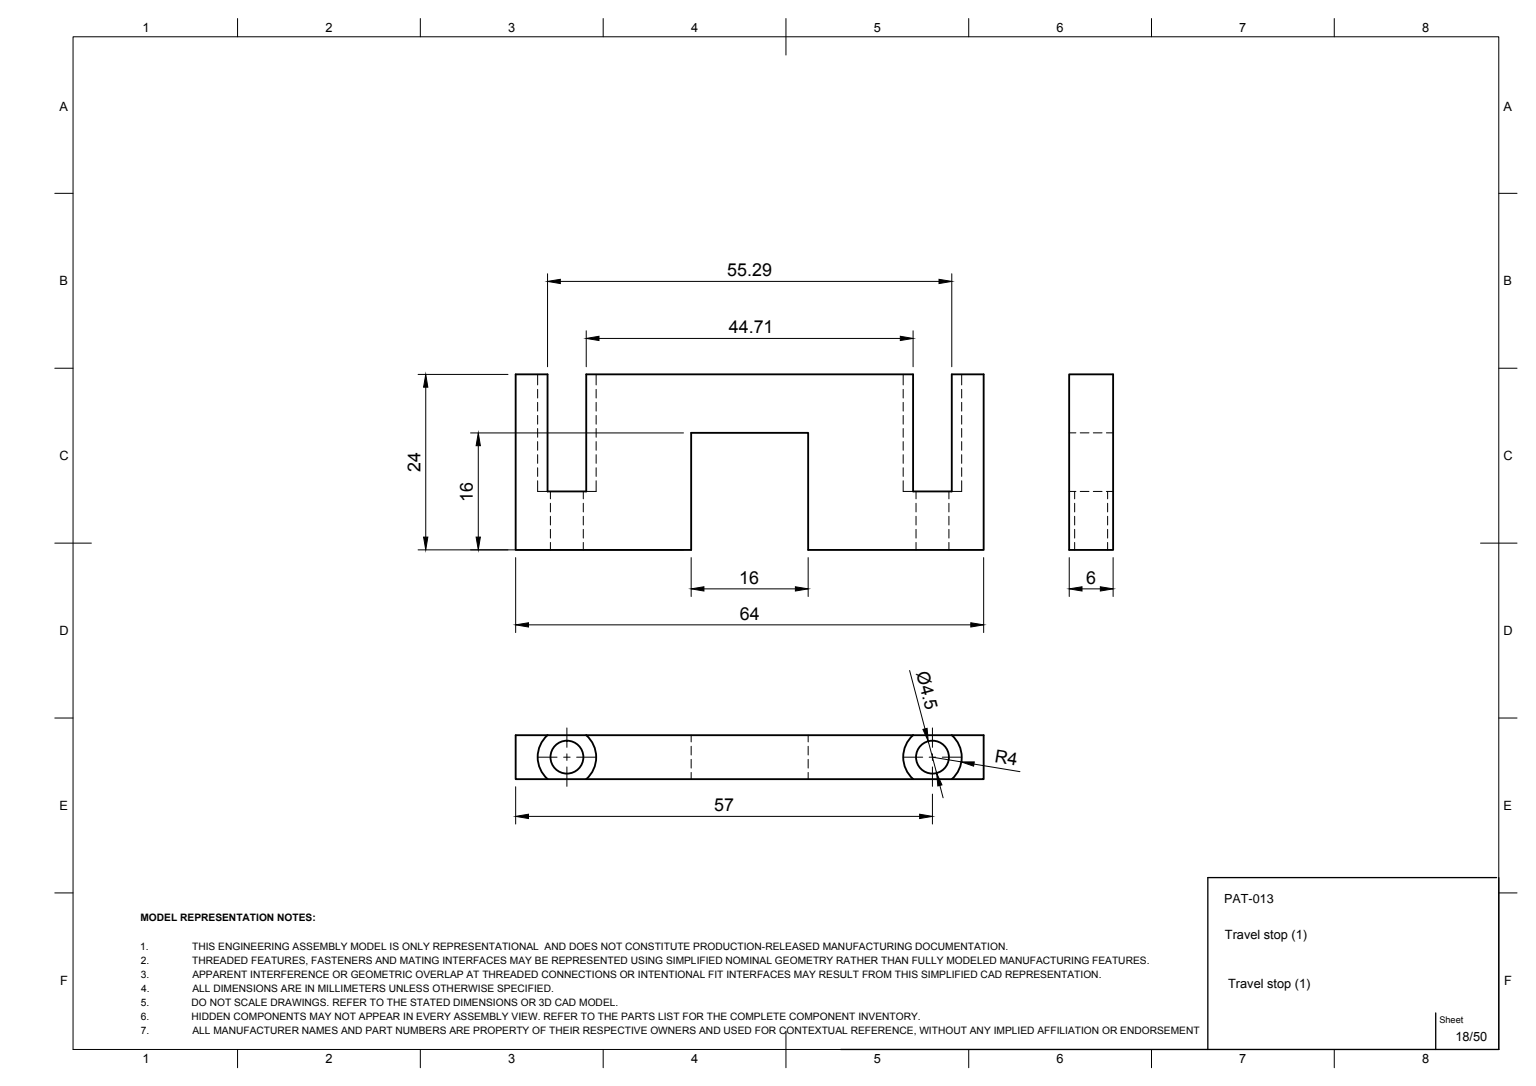
ISO-10303-21;
HEADER;
/* Generated by software containing ST-Developer
 * from STEP Tools, Inc. (www.steptools.com) 
 */

FILE_DESCRIPTION(
/* description */ ('Belt-driven linear axis on 2020 extrusion'),
/* implementation_level */ '2;1');

FILE_NAME(
/* name */ 'Travel stop (1).step',
/* time_stamp */ '2026-10-28T03:26:09-07:00',
/* author */ (''),
/* organization */ (''),
/* preprocessor_version */ 'ST-DEVELOPER v20.2',
/* originating_system */ 'Autodesk Translation Framework v15.17.0.0',
/* authorisation */ '');

FILE_SCHEMA (('AUTOMOTIVE_DESIGN { 1 0 10303 214 3 1 1 }'));
ENDSEC;

DATA;
#10=MECHANICAL_DESIGN_GEOMETRIC_PRESENTATION_REPRESENTATION('',(#625),#20096);
#531=SHAPE_REPRESENTATION_RELATIONSHIP('SRR','None',#20327,#577);
#577=ADVANCED_BREP_SHAPE_REPRESENTATION('',(#681),#20058);
#625=STYLED_ITEM('',(#20636),#681);
#681=MANIFOLD_SOLID_BREP('Body1',#10938);
#800=FACE_BOUND('',#2151,.T.);
#801=FACE_BOUND('',#2155,.T.);
#802=FACE_BOUND('',#2167,.T.);
#803=FACE_BOUND('',#2169,.T.);
#991=PLANE('',#11890);
#992=PLANE('',#11898);
#993=PLANE('',#11900);
#994=PLANE('',#11901);
#995=PLANE('',#11902);
#996=PLANE('',#11903);
#997=PLANE('',#11908);
#998=PLANE('',#11909);
#999=PLANE('',#11910);
#1000=PLANE('',#11911);
#1001=PLANE('',#11912);
#1002=PLANE('',#11913);
#1003=PLANE('',#11914);
#1004=PLANE('',#11915);
#1444=FACE_OUTER_BOUND('',#2148,.T.);
#1445=FACE_OUTER_BOUND('',#2149,.T.);
#1446=FACE_OUTER_BOUND('',#2150,.T.);
#1447=FACE_OUTER_BOUND('',#2152,.T.);
#1448=FACE_OUTER_BOUND('',#2153,.T.);
#1449=FACE_OUTER_BOUND('',#2154,.T.);
#1450=FACE_OUTER_BOUND('',#2156,.T.);
#1451=FACE_OUTER_BOUND('',#2157,.T.);
#1452=FACE_OUTER_BOUND('',#2158,.T.);
#1453=FACE_OUTER_BOUND('',#2159,.T.);
#1454=FACE_OUTER_BOUND('',#2160,.T.);
#1455=FACE_OUTER_BOUND('',#2161,.T.);
#1456=FACE_OUTER_BOUND('',#2162,.T.);
#1457=FACE_OUTER_BOUND('',#2163,.T.);
#1458=FACE_OUTER_BOUND('',#2164,.T.);
#1459=FACE_OUTER_BOUND('',#2165,.T.);
#1460=FACE_OUTER_BOUND('',#2166,.T.);
#1461=FACE_OUTER_BOUND('',#2168,.T.);
#1462=FACE_OUTER_BOUND('',#2170,.T.);
#1463=FACE_OUTER_BOUND('',#2171,.T.);
#2148=EDGE_LOOP('',(#8117,#8118,#8119,#8120));
#2149=EDGE_LOOP('',(#8121,#8122,#8123,#8124));
#2150=EDGE_LOOP('',(#8125,#8126,#8127,#8128));
#2151=EDGE_LOOP('',(#8129));
#2152=EDGE_LOOP('',(#8130,#8131,#8132,#8133));
#2153=EDGE_LOOP('',(#8134,#8135,#8136,#8137));
#2154=EDGE_LOOP('',(#8138,#8139,#8140,#8141));
#2155=EDGE_LOOP('',(#8142));
#2156=EDGE_LOOP('',(#8143,#8144,#8145,#8146,#8147,#8148,#8149,#8150,#8151,
#8152,#8153,#8154,#8155,#8156,#8157,#8158));
#2157=EDGE_LOOP('',(#8159,#8160,#8161,#8162));
#2158=EDGE_LOOP('',(#8163,#8164,#8165,#8166));
#2159=EDGE_LOOP('',(#8167,#8168,#8169,#8170));
#2160=EDGE_LOOP('',(#8171,#8172,#8173,#8174));
#2161=EDGE_LOOP('',(#8175,#8176,#8177,#8178));
#2162=EDGE_LOOP('',(#8179,#8180,#8181,#8182));
#2163=EDGE_LOOP('',(#8183,#8184,#8185,#8186));
#2164=EDGE_LOOP('',(#8187,#8188,#8189,#8190));
#2165=EDGE_LOOP('',(#8191,#8192,#8193,#8194,#8195,#8196,#8197,#8198,#8199,
#8200,#8201,#8202,#8203,#8204,#8205,#8206));
#2166=EDGE_LOOP('',(#8207,#8208,#8209,#8210));
#2167=EDGE_LOOP('',(#8211));
#2168=EDGE_LOOP('',(#8212,#8213,#8214,#8215));
#2169=EDGE_LOOP('',(#8216));
#2170=EDGE_LOOP('',(#8217,#8218,#8219,#8220));
#2171=EDGE_LOOP('',(#8221,#8222,#8223,#8224));
#2913=LINE('',#17165,#3770);
#2914=LINE('',#17169,#3771);
#2915=LINE('',#17174,#3772);
#2916=LINE('',#17178,#3773);
#2917=LINE('',#17181,#3774);
#2918=LINE('',#17182,#3775);
#2919=LINE('',#17188,#3776);
#2920=LINE('',#17192,#3777);
#2921=LINE('',#17197,#3778);
#2922=LINE('',#17201,#3779);
#2923=LINE('',#17204,#3780);
#2924=LINE('',#17205,#3781);
#2925=LINE('',#17210,#3782);
#2926=LINE('',#17212,#3783);
#2927=LINE('',#17214,#3784);
#2928=LINE('',#17216,#3785);
#2929=LINE('',#17218,#3786);
#2930=LINE('',#17220,#3787);
#2931=LINE('',#17222,#3788);
#2932=LINE('',#17224,#3789);
#2933=LINE('',#17225,#3790);
#2934=LINE('',#17226,#3791);
#2935=LINE('',#17229,#3792);
#2936=LINE('',#17230,#3793);
#2937=LINE('',#17233,#3794);
#2938=LINE('',#17234,#3795);
#2939=LINE('',#17236,#3796);
#2940=LINE('',#17240,#3797);
#2941=LINE('',#17244,#3798);
#2942=LINE('',#17247,#3799);
#2943=LINE('',#17249,#3800);
#2944=LINE('',#17250,#3801);
#2945=LINE('',#17253,#3802);
#2946=LINE('',#17255,#3803);
#2947=LINE('',#17256,#3804);
#2948=LINE('',#17258,#3805);
#2949=LINE('',#17261,#3806);
#2950=LINE('',#17262,#3807);
#2951=LINE('',#17264,#3808);
#2952=LINE('',#17265,#3809);
#2953=LINE('',#17267,#3810);
#2954=LINE('',#17269,#3811);
#3770=VECTOR('',#13823,1.);
#3771=VECTOR('',#13826,1.);
#3772=VECTOR('',#13831,1.);
#3773=VECTOR('',#13834,1.);
#3774=VECTOR('',#13839,1.);
#3775=VECTOR('',#13840,1.);
#3776=VECTOR('',#13845,1.);
#3777=VECTOR('',#13848,1.);
#3778=VECTOR('',#13853,1.);
#3779=VECTOR('',#13856,1.);
#3780=VECTOR('',#13861,1.);
#3781=VECTOR('',#13862,1.);
#3782=VECTOR('',#13867,1.);
#3783=VECTOR('',#13868,1.);
#3784=VECTOR('',#13869,1.);
#3785=VECTOR('',#13870,1.);
#3786=VECTOR('',#13871,1.);
#3787=VECTOR('',#13872,1.);
#3788=VECTOR('',#13873,1.);
#3789=VECTOR('',#13874,1.);
#3790=VECTOR('',#13875,1.);
#3791=VECTOR('',#13876,1.);
#3792=VECTOR('',#13879,1.);
#3793=VECTOR('',#13880,1.);
#3794=VECTOR('',#13883,1.);
#3795=VECTOR('',#13884,1.);
#3796=VECTOR('',#13887,1.);
#3797=VECTOR('',#13892,0.225000000000001);
#3798=VECTOR('',#13897,0.225000000000001);
#3799=VECTOR('',#13900,1.);
#3800=VECTOR('',#13901,1.);
#3801=VECTOR('',#13902,1.);
#3802=VECTOR('',#13905,1.);
#3803=VECTOR('',#13906,1.);
#3804=VECTOR('',#13907,1.);
#3805=VECTOR('',#13910,1.);
#3806=VECTOR('',#13913,1.);
#3807=VECTOR('',#13914,1.);
#3808=VECTOR('',#13915,1.);
#3809=VECTOR('',#13916,1.);
#3810=VECTOR('',#13919,1.);
#3811=VECTOR('',#13922,1.);
#4563=CIRCLE('',#11885,0.399999999999999);
#4564=CIRCLE('',#11886,0.399999999999999);
#4565=CIRCLE('',#11888,0.399999999999999);
#4566=CIRCLE('',#11889,0.399999999999999);
#4567=CIRCLE('',#11891,0.225000000000001);
#4568=CIRCLE('',#11893,0.399999999999999);
#4569=CIRCLE('',#11894,0.399999999999999);
#4570=CIRCLE('',#11896,0.399999999999999);
#4571=CIRCLE('',#11897,0.399999999999999);
#4572=CIRCLE('',#11899,0.225000000000001);
#4573=CIRCLE('',#11905,0.225000000000001);
#4574=CIRCLE('',#11907,0.225000000000001);
#5180=VERTEX_POINT('',#17163);
#5181=VERTEX_POINT('',#17164);
#5182=VERTEX_POINT('',#17166);
#5183=VERTEX_POINT('',#17168);
#5184=VERTEX_POINT('',#17172);
#5185=VERTEX_POINT('',#17173);
#5186=VERTEX_POINT('',#17175);
#5187=VERTEX_POINT('',#17177);
#5188=VERTEX_POINT('',#17183);
#5189=VERTEX_POINT('',#17186);
#5190=VERTEX_POINT('',#17187);
#5191=VERTEX_POINT('',#17189);
#5192=VERTEX_POINT('',#17191);
#5193=VERTEX_POINT('',#17195);
#5194=VERTEX_POINT('',#17196);
#5195=VERTEX_POINT('',#17198);
#5196=VERTEX_POINT('',#17200);
#5197=VERTEX_POINT('',#17206);
#5198=VERTEX_POINT('',#17209);
#5199=VERTEX_POINT('',#17211);
#5200=VERTEX_POINT('',#17213);
#5201=VERTEX_POINT('',#17215);
#5202=VERTEX_POINT('',#17217);
#5203=VERTEX_POINT('',#17219);
#5204=VERTEX_POINT('',#17221);
#5205=VERTEX_POINT('',#17223);
#5206=VERTEX_POINT('',#17228);
#5207=VERTEX_POINT('',#17232);
#5208=VERTEX_POINT('',#17238);
#5209=VERTEX_POINT('',#17242);
#5210=VERTEX_POINT('',#17246);
#5211=VERTEX_POINT('',#17248);
#5212=VERTEX_POINT('',#17252);
#5213=VERTEX_POINT('',#17254);
#5214=VERTEX_POINT('',#17260);
#5215=VERTEX_POINT('',#17263);
#6273=EDGE_CURVE('',#5180,#5181,#2913,.T.);
#6274=EDGE_CURVE('',#5182,#5180,#4563,.T.);
#6275=EDGE_CURVE('',#5183,#5182,#2914,.T.);
#6276=EDGE_CURVE('',#5181,#5183,#4564,.T.);
#6277=EDGE_CURVE('',#5184,#5185,#2915,.T.);
#6278=EDGE_CURVE('',#5186,#5184,#4565,.T.);
#6279=EDGE_CURVE('',#5187,#5186,#2916,.T.);
#6280=EDGE_CURVE('',#5185,#5187,#4566,.T.);
#6281=EDGE_CURVE('',#5181,#5184,#2917,.T.);
#6282=EDGE_CURVE('',#5186,#5183,#2918,.T.);
#6283=EDGE_CURVE('',#5188,#5188,#4567,.T.);
#6284=EDGE_CURVE('',#5189,#5190,#2919,.T.);
#6285=EDGE_CURVE('',#5191,#5189,#4568,.T.);
#6286=EDGE_CURVE('',#5192,#5191,#2920,.T.);
#6287=EDGE_CURVE('',#5190,#5192,#4569,.T.);
#6288=EDGE_CURVE('',#5193,#5194,#2921,.T.);
#6289=EDGE_CURVE('',#5195,#5193,#4570,.T.);
#6290=EDGE_CURVE('',#5196,#5195,#2922,.T.);
#6291=EDGE_CURVE('',#5194,#5196,#4571,.T.);
#6292=EDGE_CURVE('',#5190,#5193,#2923,.T.);
#6293=EDGE_CURVE('',#5195,#5192,#2924,.T.);
#6294=EDGE_CURVE('',#5197,#5197,#4572,.T.);
#6295=EDGE_CURVE('',#5198,#5182,#2925,.T.);
#6296=EDGE_CURVE('',#5199,#5198,#2926,.T.);
#6297=EDGE_CURVE('',#5199,#5200,#2927,.T.);
#6298=EDGE_CURVE('',#5200,#5201,#2928,.T.);
#6299=EDGE_CURVE('',#5201,#5202,#2929,.T.);
#6300=EDGE_CURVE('',#5202,#5203,#2930,.T.);
#6301=EDGE_CURVE('',#5203,#5204,#2931,.T.);
#6302=EDGE_CURVE('',#5204,#5205,#2932,.T.);
#6303=EDGE_CURVE('',#5196,#5205,#2933,.T.);
#6304=EDGE_CURVE('',#5187,#5191,#2934,.T.);
#6305=EDGE_CURVE('',#5205,#5206,#2935,.T.);
#6306=EDGE_CURVE('',#5206,#5194,#2936,.T.);
#6307=EDGE_CURVE('',#5180,#5207,#2937,.T.);
#6308=EDGE_CURVE('',#5207,#5198,#2938,.T.);
#6309=EDGE_CURVE('',#5189,#5185,#2939,.T.);
#6310=EDGE_CURVE('',#5208,#5208,#4573,.T.);
#6311=EDGE_CURVE('',#5208,#5188,#2940,.T.);
#6312=EDGE_CURVE('',#5209,#5209,#4574,.T.);
#6313=EDGE_CURVE('',#5209,#5197,#2941,.T.);
#6314=EDGE_CURVE('',#5202,#5210,#2942,.T.);
#6315=EDGE_CURVE('',#5211,#5210,#2943,.T.);
#6316=EDGE_CURVE('',#5203,#5211,#2944,.T.);
#6317=EDGE_CURVE('',#5212,#5200,#2945,.T.);
#6318=EDGE_CURVE('',#5213,#5212,#2946,.T.);
#6319=EDGE_CURVE('',#5213,#5201,#2947,.T.);
#6320=EDGE_CURVE('',#5210,#5213,#2948,.T.);
#6321=EDGE_CURVE('',#5214,#5206,#2949,.T.);
#6322=EDGE_CURVE('',#5214,#5211,#2950,.T.);
#6323=EDGE_CURVE('',#5212,#5215,#2951,.T.);
#6324=EDGE_CURVE('',#5215,#5207,#2952,.T.);
#6325=EDGE_CURVE('',#5215,#5199,#2953,.T.);
#6326=EDGE_CURVE('',#5204,#5214,#2954,.T.);
#8117=ORIENTED_EDGE('',*,*,#6273,.F.);
#8118=ORIENTED_EDGE('',*,*,#6274,.F.);
#8119=ORIENTED_EDGE('',*,*,#6275,.F.);
#8120=ORIENTED_EDGE('',*,*,#6276,.F.);
#8121=ORIENTED_EDGE('',*,*,#6277,.F.);
#8122=ORIENTED_EDGE('',*,*,#6278,.F.);
#8123=ORIENTED_EDGE('',*,*,#6279,.F.);
#8124=ORIENTED_EDGE('',*,*,#6280,.F.);
#8125=ORIENTED_EDGE('',*,*,#6281,.F.);
#8126=ORIENTED_EDGE('',*,*,#6276,.T.);
#8127=ORIENTED_EDGE('',*,*,#6282,.F.);
#8128=ORIENTED_EDGE('',*,*,#6278,.T.);
#8129=ORIENTED_EDGE('',*,*,#6283,.F.);
#8130=ORIENTED_EDGE('',*,*,#6284,.F.);
#8131=ORIENTED_EDGE('',*,*,#6285,.F.);
#8132=ORIENTED_EDGE('',*,*,#6286,.F.);
#8133=ORIENTED_EDGE('',*,*,#6287,.F.);
#8134=ORIENTED_EDGE('',*,*,#6288,.F.);
#8135=ORIENTED_EDGE('',*,*,#6289,.F.);
#8136=ORIENTED_EDGE('',*,*,#6290,.F.);
#8137=ORIENTED_EDGE('',*,*,#6291,.F.);
#8138=ORIENTED_EDGE('',*,*,#6292,.F.);
#8139=ORIENTED_EDGE('',*,*,#6287,.T.);
#8140=ORIENTED_EDGE('',*,*,#6293,.F.);
#8141=ORIENTED_EDGE('',*,*,#6289,.T.);
#8142=ORIENTED_EDGE('',*,*,#6294,.F.);
#8143=ORIENTED_EDGE('',*,*,#6279,.T.);
#8144=ORIENTED_EDGE('',*,*,#6282,.T.);
#8145=ORIENTED_EDGE('',*,*,#6275,.T.);
#8146=ORIENTED_EDGE('',*,*,#6295,.F.);
#8147=ORIENTED_EDGE('',*,*,#6296,.F.);
#8148=ORIENTED_EDGE('',*,*,#6297,.T.);
#8149=ORIENTED_EDGE('',*,*,#6298,.T.);
#8150=ORIENTED_EDGE('',*,*,#6299,.T.);
#8151=ORIENTED_EDGE('',*,*,#6300,.T.);
#8152=ORIENTED_EDGE('',*,*,#6301,.T.);
#8153=ORIENTED_EDGE('',*,*,#6302,.T.);
#8154=ORIENTED_EDGE('',*,*,#6303,.F.);
#8155=ORIENTED_EDGE('',*,*,#6290,.T.);
#8156=ORIENTED_EDGE('',*,*,#6293,.T.);
#8157=ORIENTED_EDGE('',*,*,#6286,.T.);
#8158=ORIENTED_EDGE('',*,*,#6304,.F.);
#8159=ORIENTED_EDGE('',*,*,#6291,.T.);
#8160=ORIENTED_EDGE('',*,*,#6303,.T.);
#8161=ORIENTED_EDGE('',*,*,#6305,.T.);
#8162=ORIENTED_EDGE('',*,*,#6306,.T.);
#8163=ORIENTED_EDGE('',*,*,#6274,.T.);
#8164=ORIENTED_EDGE('',*,*,#6307,.T.);
#8165=ORIENTED_EDGE('',*,*,#6308,.T.);
#8166=ORIENTED_EDGE('',*,*,#6295,.T.);
#8167=ORIENTED_EDGE('',*,*,#6280,.T.);
#8168=ORIENTED_EDGE('',*,*,#6304,.T.);
#8169=ORIENTED_EDGE('',*,*,#6285,.T.);
#8170=ORIENTED_EDGE('',*,*,#6309,.T.);
#8171=ORIENTED_EDGE('',*,*,#6310,.F.);
#8172=ORIENTED_EDGE('',*,*,#6311,.T.);
#8173=ORIENTED_EDGE('',*,*,#6283,.T.);
#8174=ORIENTED_EDGE('',*,*,#6311,.F.);
#8175=ORIENTED_EDGE('',*,*,#6312,.F.);
#8176=ORIENTED_EDGE('',*,*,#6313,.T.);
#8177=ORIENTED_EDGE('',*,*,#6294,.T.);
#8178=ORIENTED_EDGE('',*,*,#6313,.F.);
#8179=ORIENTED_EDGE('',*,*,#6300,.F.);
#8180=ORIENTED_EDGE('',*,*,#6314,.T.);
#8181=ORIENTED_EDGE('',*,*,#6315,.F.);
#8182=ORIENTED_EDGE('',*,*,#6316,.F.);
#8183=ORIENTED_EDGE('',*,*,#6298,.F.);
#8184=ORIENTED_EDGE('',*,*,#6317,.F.);
#8185=ORIENTED_EDGE('',*,*,#6318,.F.);
#8186=ORIENTED_EDGE('',*,*,#6319,.T.);
#8187=ORIENTED_EDGE('',*,*,#6299,.F.);
#8188=ORIENTED_EDGE('',*,*,#6319,.F.);
#8189=ORIENTED_EDGE('',*,*,#6320,.F.);
#8190=ORIENTED_EDGE('',*,*,#6314,.F.);
#8191=ORIENTED_EDGE('',*,*,#6277,.T.);
#8192=ORIENTED_EDGE('',*,*,#6309,.F.);
#8193=ORIENTED_EDGE('',*,*,#6284,.T.);
#8194=ORIENTED_EDGE('',*,*,#6292,.T.);
#8195=ORIENTED_EDGE('',*,*,#6288,.T.);
#8196=ORIENTED_EDGE('',*,*,#6306,.F.);
#8197=ORIENTED_EDGE('',*,*,#6321,.F.);
#8198=ORIENTED_EDGE('',*,*,#6322,.T.);
#8199=ORIENTED_EDGE('',*,*,#6315,.T.);
#8200=ORIENTED_EDGE('',*,*,#6320,.T.);
#8201=ORIENTED_EDGE('',*,*,#6318,.T.);
#8202=ORIENTED_EDGE('',*,*,#6323,.T.);
#8203=ORIENTED_EDGE('',*,*,#6324,.T.);
#8204=ORIENTED_EDGE('',*,*,#6307,.F.);
#8205=ORIENTED_EDGE('',*,*,#6273,.T.);
#8206=ORIENTED_EDGE('',*,*,#6281,.T.);
#8207=ORIENTED_EDGE('',*,*,#6317,.T.);
#8208=ORIENTED_EDGE('',*,*,#6297,.F.);
#8209=ORIENTED_EDGE('',*,*,#6325,.F.);
#8210=ORIENTED_EDGE('',*,*,#6323,.F.);
#8211=ORIENTED_EDGE('',*,*,#6310,.T.);
#8212=ORIENTED_EDGE('',*,*,#6316,.T.);
#8213=ORIENTED_EDGE('',*,*,#6322,.F.);
#8214=ORIENTED_EDGE('',*,*,#6326,.F.);
#8215=ORIENTED_EDGE('',*,*,#6301,.F.);
#8216=ORIENTED_EDGE('',*,*,#6312,.T.);
#8217=ORIENTED_EDGE('',*,*,#6326,.T.);
#8218=ORIENTED_EDGE('',*,*,#6321,.T.);
#8219=ORIENTED_EDGE('',*,*,#6305,.F.);
#8220=ORIENTED_EDGE('',*,*,#6302,.F.);
#8221=ORIENTED_EDGE('',*,*,#6325,.T.);
#8222=ORIENTED_EDGE('',*,*,#6296,.T.);
#8223=ORIENTED_EDGE('',*,*,#6308,.F.);
#8224=ORIENTED_EDGE('',*,*,#6324,.F.);
#10169=CYLINDRICAL_SURFACE('',#11884,0.399999999999999);
#10170=CYLINDRICAL_SURFACE('',#11887,0.399999999999999);
#10171=CYLINDRICAL_SURFACE('',#11892,0.399999999999999);
#10172=CYLINDRICAL_SURFACE('',#11895,0.399999999999999);
#10173=CYLINDRICAL_SURFACE('',#11904,0.225000000000001);
#10174=CYLINDRICAL_SURFACE('',#11906,0.225000000000001);
#10495=ADVANCED_FACE('',(#1444),#10169,.F.);
#10496=ADVANCED_FACE('',(#1445),#10170,.F.);
#10497=ADVANCED_FACE('',(#1446,#800),#991,.T.);
#10498=ADVANCED_FACE('',(#1447),#10171,.F.);
#10499=ADVANCED_FACE('',(#1448),#10172,.F.);
#10500=ADVANCED_FACE('',(#1449,#801),#992,.T.);
#10501=ADVANCED_FACE('',(#1450),#993,.T.);
#10502=ADVANCED_FACE('',(#1451),#994,.T.);
#10503=ADVANCED_FACE('',(#1452),#995,.T.);
#10504=ADVANCED_FACE('',(#1453),#996,.T.);
#10505=ADVANCED_FACE('',(#1454),#10173,.F.);
#10506=ADVANCED_FACE('',(#1455),#10174,.F.);
#10507=ADVANCED_FACE('',(#1456),#997,.F.);
#10508=ADVANCED_FACE('',(#1457),#998,.F.);
#10509=ADVANCED_FACE('',(#1458),#999,.F.);
#10510=ADVANCED_FACE('',(#1459),#1000,.T.);
#10511=ADVANCED_FACE('',(#1460,#802),#1001,.F.);
#10512=ADVANCED_FACE('',(#1461,#803),#1002,.F.);
#10513=ADVANCED_FACE('',(#1462),#1003,.T.);
#10514=ADVANCED_FACE('',(#1463),#1004,.T.);
#10938=CLOSED_SHELL('',(#10495,#10496,#10497,#10498,#10499,#10500,#10501,
#10502,#10503,#10504,#10505,#10506,#10507,#10508,#10509,#10510,#10511,#10512,
#10513,#10514));
#11883=AXIS2_PLACEMENT_3D('',#17161,#13819,#13820);
#11884=AXIS2_PLACEMENT_3D('',#17162,#13821,#13822);
#11885=AXIS2_PLACEMENT_3D('',#17167,#13824,#13825);
#11886=AXIS2_PLACEMENT_3D('',#17170,#13827,#13828);
#11887=AXIS2_PLACEMENT_3D('',#17171,#13829,#13830);
#11888=AXIS2_PLACEMENT_3D('',#17176,#13832,#13833);
#11889=AXIS2_PLACEMENT_3D('',#17179,#13835,#13836);
#11890=AXIS2_PLACEMENT_3D('',#17180,#13837,#13838);
#11891=AXIS2_PLACEMENT_3D('',#17184,#13841,#13842);
#11892=AXIS2_PLACEMENT_3D('',#17185,#13843,#13844);
#11893=AXIS2_PLACEMENT_3D('',#17190,#13846,#13847);
#11894=AXIS2_PLACEMENT_3D('',#17193,#13849,#13850);
#11895=AXIS2_PLACEMENT_3D('',#17194,#13851,#13852);
#11896=AXIS2_PLACEMENT_3D('',#17199,#13854,#13855);
#11897=AXIS2_PLACEMENT_3D('',#17202,#13857,#13858);
#11898=AXIS2_PLACEMENT_3D('',#17203,#13859,#13860);
#11899=AXIS2_PLACEMENT_3D('',#17207,#13863,#13864);
#11900=AXIS2_PLACEMENT_3D('',#17208,#13865,#13866);
#11901=AXIS2_PLACEMENT_3D('',#17227,#13877,#13878);
#11902=AXIS2_PLACEMENT_3D('',#17231,#13881,#13882);
#11903=AXIS2_PLACEMENT_3D('',#17235,#13885,#13886);
#11904=AXIS2_PLACEMENT_3D('',#17237,#13888,#13889);
#11905=AXIS2_PLACEMENT_3D('',#17239,#13890,#13891);
#11906=AXIS2_PLACEMENT_3D('',#17241,#13893,#13894);
#11907=AXIS2_PLACEMENT_3D('',#17243,#13895,#13896);
#11908=AXIS2_PLACEMENT_3D('',#17245,#13898,#13899);
#11909=AXIS2_PLACEMENT_3D('',#17251,#13903,#13904);
#11910=AXIS2_PLACEMENT_3D('',#17257,#13908,#13909);
#11911=AXIS2_PLACEMENT_3D('',#17259,#13911,#13912);
#11912=AXIS2_PLACEMENT_3D('',#17266,#13917,#13918);
#11913=AXIS2_PLACEMENT_3D('',#17268,#13920,#13921);
#11914=AXIS2_PLACEMENT_3D('',#17270,#13923,#13924);
#11915=AXIS2_PLACEMENT_3D('',#17271,#13925,#13926);
#13819=DIRECTION('axis',(0.,0.,1.));
#13820=DIRECTION('refdir',(1.,0.,0.));
#13821=DIRECTION('center_axis',(0.,0.,1.));
#13822=DIRECTION('ref_axis',(1.,0.,0.));
#13823=DIRECTION('',(0.,0.,-1.));
#13824=DIRECTION('center_axis',(0.,0.,-1.));
#13825=DIRECTION('ref_axis',(1.,0.,0.));
#13826=DIRECTION('',(0.,0.,1.));
#13827=DIRECTION('center_axis',(0.,0.,1.));
#13828=DIRECTION('ref_axis',(1.,0.,0.));
#13829=DIRECTION('center_axis',(0.,0.,1.));
#13830=DIRECTION('ref_axis',(1.,0.,0.));
#13831=DIRECTION('',(0.,0.,1.));
#13832=DIRECTION('center_axis',(0.,0.,1.));
#13833=DIRECTION('ref_axis',(1.,0.,0.));
#13834=DIRECTION('',(0.,0.,-1.));
#13835=DIRECTION('center_axis',(0.,0.,-1.));
#13836=DIRECTION('ref_axis',(1.,0.,0.));
#13837=DIRECTION('center_axis',(0.,0.,1.));
#13838=DIRECTION('ref_axis',(1.,0.,0.));
#13839=DIRECTION('',(0.,1.,0.));
#13840=DIRECTION('',(0.,-1.,0.));
#13841=DIRECTION('center_axis',(0.,0.,1.));
#13842=DIRECTION('ref_axis',(1.,0.,0.));
#13843=DIRECTION('center_axis',(0.,0.,1.));
#13844=DIRECTION('ref_axis',(1.,0.,0.));
#13845=DIRECTION('',(0.,0.,-1.));
#13846=DIRECTION('center_axis',(0.,0.,-1.));
#13847=DIRECTION('ref_axis',(1.,0.,0.));
#13848=DIRECTION('',(0.,0.,1.));
#13849=DIRECTION('center_axis',(0.,0.,1.));
#13850=DIRECTION('ref_axis',(1.,0.,0.));
#13851=DIRECTION('center_axis',(0.,0.,1.));
#13852=DIRECTION('ref_axis',(1.,0.,0.));
#13853=DIRECTION('',(0.,0.,1.));
#13854=DIRECTION('center_axis',(0.,0.,1.));
#13855=DIRECTION('ref_axis',(1.,0.,0.));
#13856=DIRECTION('',(0.,0.,-1.));
#13857=DIRECTION('center_axis',(0.,0.,-1.));
#13858=DIRECTION('ref_axis',(1.,0.,0.));
#13859=DIRECTION('center_axis',(0.,0.,1.));
#13860=DIRECTION('ref_axis',(1.,0.,0.));
#13861=DIRECTION('',(0.,1.,0.));
#13862=DIRECTION('',(0.,-1.,0.));
#13863=DIRECTION('center_axis',(0.,0.,1.));
#13864=DIRECTION('ref_axis',(1.,0.,0.));
#13865=DIRECTION('center_axis',(1.,0.,0.));
#13866=DIRECTION('ref_axis',(0.,1.,0.));
#13867=DIRECTION('',(0.,1.,0.));
#13868=DIRECTION('',(0.,0.,1.));
#13869=DIRECTION('',(0.,1.,0.));
#13870=DIRECTION('',(0.,0.,1.));
#13871=DIRECTION('',(0.,1.,0.));
#13872=DIRECTION('',(0.,0.,-1.));
#13873=DIRECTION('',(0.,1.,0.));
#13874=DIRECTION('',(0.,0.,1.));
#13875=DIRECTION('',(0.,1.,0.));
#13876=DIRECTION('',(0.,1.,0.));
#13877=DIRECTION('center_axis',(0.,0.,1.));
#13878=DIRECTION('ref_axis',(1.,0.,0.));
#13879=DIRECTION('',(-1.,0.,0.));
#13880=DIRECTION('',(0.,-1.,0.));
#13881=DIRECTION('center_axis',(0.,0.,1.));
#13882=DIRECTION('ref_axis',(1.,0.,0.));
#13883=DIRECTION('',(0.,-1.,0.));
#13884=DIRECTION('',(1.,0.,0.));
#13885=DIRECTION('center_axis',(0.,0.,1.));
#13886=DIRECTION('ref_axis',(1.,0.,0.));
#13887=DIRECTION('',(0.,-1.,0.));
#13888=DIRECTION('center_axis',(0.,0.,1.));
#13889=DIRECTION('ref_axis',(1.,0.,0.));
#13890=DIRECTION('center_axis',(0.,0.,1.));
#13891=DIRECTION('ref_axis',(1.,0.,0.));
#13892=DIRECTION('',(0.,0.,1.));
#13893=DIRECTION('center_axis',(0.,0.,1.));
#13894=DIRECTION('ref_axis',(1.,0.,0.));
#13895=DIRECTION('center_axis',(0.,0.,1.));
#13896=DIRECTION('ref_axis',(1.,0.,0.));
#13897=DIRECTION('',(0.,0.,1.));
#13898=DIRECTION('center_axis',(0.,1.,0.));
#13899=DIRECTION('ref_axis',(-1.,0.,0.));
#13900=DIRECTION('',(-1.,0.,0.));
#13901=DIRECTION('',(0.,0.,1.));
#13902=DIRECTION('',(-1.,0.,0.));
#13903=DIRECTION('center_axis',(0.,-1.,0.));
#13904=DIRECTION('ref_axis',(1.,0.,0.));
#13905=DIRECTION('',(1.,0.,0.));
#13906=DIRECTION('',(0.,0.,-1.));
#13907=DIRECTION('',(1.,0.,0.));
#13908=DIRECTION('center_axis',(0.,0.,1.));
#13909=DIRECTION('ref_axis',(1.,0.,0.));
#13910=DIRECTION('',(0.,-1.,0.));
#13911=DIRECTION('center_axis',(-1.,0.,0.));
#13912=DIRECTION('ref_axis',(0.,-1.,0.));
#13913=DIRECTION('',(0.,0.,1.));
#13914=DIRECTION('',(0.,-1.,0.));
#13915=DIRECTION('',(0.,-1.,0.));
#13916=DIRECTION('',(0.,0.,1.));
#13917=DIRECTION('center_axis',(0.,0.,1.));
#13918=DIRECTION('ref_axis',(1.,0.,0.));
#13919=DIRECTION('',(1.,0.,0.));
#13920=DIRECTION('center_axis',(0.,0.,1.));
#13921=DIRECTION('ref_axis',(1.,0.,0.));
#13922=DIRECTION('',(-1.,0.,0.));
#13923=DIRECTION('center_axis',(0.,1.,0.));
#13924=DIRECTION('ref_axis',(-1.,0.,0.));
#13925=DIRECTION('center_axis',(0.,-1.,0.));
#13926=DIRECTION('ref_axis',(1.,0.,0.));
#17161=CARTESIAN_POINT('',(0.,0.,0.));
#17162=CARTESIAN_POINT('Origin',(26.2,-2.5,0.8));
#17163=CARTESIAN_POINT('',(25.9,-2.76457513110646,2.4));
#17164=CARTESIAN_POINT('',(25.9,-2.76457513110646,0.8));
#17165=CARTESIAN_POINT('',(25.9,-2.76457513110646,0.8));
#17166=CARTESIAN_POINT('',(26.5,-2.76457513110646,2.4));
#17167=CARTESIAN_POINT('Origin',(26.2,-2.5,2.4));
#17168=CARTESIAN_POINT('',(26.5,-2.76457513110646,0.8));
#17169=CARTESIAN_POINT('',(26.5,-2.76457513110646,0.8));
#17170=CARTESIAN_POINT('Origin',(26.2,-2.5,0.8));
#17171=CARTESIAN_POINT('Origin',(26.2,-2.5,0.8));
#17172=CARTESIAN_POINT('',(25.9,-2.23542486889354,0.8));
#17173=CARTESIAN_POINT('',(25.9,-2.23542486889354,2.4));
#17174=CARTESIAN_POINT('',(25.9,-2.23542486889354,0.8));
#17175=CARTESIAN_POINT('',(26.5,-2.23542486889354,0.8));
#17176=CARTESIAN_POINT('Origin',(26.2,-2.5,0.8));
#17177=CARTESIAN_POINT('',(26.5,-2.23542486889354,2.4));
#17178=CARTESIAN_POINT('',(26.5,-2.23542486889354,0.8));
#17179=CARTESIAN_POINT('Origin',(26.2,-2.5,2.4));
#17180=CARTESIAN_POINT('Origin',(26.2,-2.5,0.8));
#17181=CARTESIAN_POINT('',(25.9,0.35,0.8));
#17182=CARTESIAN_POINT('',(26.5,-2.85,0.8));
#17183=CARTESIAN_POINT('',(25.975,-2.5,0.8));
#17184=CARTESIAN_POINT('Origin',(26.2,-2.5,0.8));
#17185=CARTESIAN_POINT('Origin',(26.2,2.5,0.8));
#17186=CARTESIAN_POINT('',(25.9,2.23542486889354,2.4));
#17187=CARTESIAN_POINT('',(25.9,2.23542486889354,0.8));
#17188=CARTESIAN_POINT('',(25.9,2.23542486889354,0.8));
#17189=CARTESIAN_POINT('',(26.5,2.23542486889354,2.4));
#17190=CARTESIAN_POINT('Origin',(26.2,2.5,2.4));
#17191=CARTESIAN_POINT('',(26.5,2.23542486889354,0.8));
#17192=CARTESIAN_POINT('',(26.5,2.23542486889354,0.8));
#17193=CARTESIAN_POINT('Origin',(26.2,2.5,0.8));
#17194=CARTESIAN_POINT('Origin',(26.2,2.5,0.8));
#17195=CARTESIAN_POINT('',(25.9,2.76457513110646,0.8));
#17196=CARTESIAN_POINT('',(25.9,2.76457513110646,2.4));
#17197=CARTESIAN_POINT('',(25.9,2.76457513110646,0.8));
#17198=CARTESIAN_POINT('',(26.5,2.76457513110646,0.8));
#17199=CARTESIAN_POINT('Origin',(26.2,2.5,0.8));
#17200=CARTESIAN_POINT('',(26.5,2.76457513110646,2.4));
#17201=CARTESIAN_POINT('',(26.5,2.76457513110646,0.8));
#17202=CARTESIAN_POINT('Origin',(26.2,2.5,2.4));
#17203=CARTESIAN_POINT('Origin',(26.2,2.5,0.8));
#17204=CARTESIAN_POINT('',(25.9,2.85,0.8));
#17205=CARTESIAN_POINT('',(26.5,-0.35,0.8));
#17206=CARTESIAN_POINT('',(25.975,2.5,0.8));
#17207=CARTESIAN_POINT('Origin',(26.2,2.5,0.8));
#17208=CARTESIAN_POINT('Origin',(26.5,-3.2,0.));
#17209=CARTESIAN_POINT('',(26.5,-3.2,2.4));
#17210=CARTESIAN_POINT('',(26.5,-3.2,2.4));
#17211=CARTESIAN_POINT('',(26.5,-3.2,0.));
#17212=CARTESIAN_POINT('',(26.5,-3.2,0.));
#17213=CARTESIAN_POINT('',(26.5,-0.8,0.));
#17214=CARTESIAN_POINT('',(26.5,-3.2,0.));
#17215=CARTESIAN_POINT('',(26.5,-0.8,1.6));
#17216=CARTESIAN_POINT('',(26.5,-0.8,-0.05));
#17217=CARTESIAN_POINT('',(26.5,0.8,1.6));
#17218=CARTESIAN_POINT('',(26.5,-1.6,1.6));
#17219=CARTESIAN_POINT('',(26.5,0.8,0.));
#17220=CARTESIAN_POINT('',(26.5,0.8,-0.05));
#17221=CARTESIAN_POINT('',(26.5,3.2,0.));
#17222=CARTESIAN_POINT('',(26.5,-3.2,0.));
#17223=CARTESIAN_POINT('',(26.5,3.2,2.4));
#17224=CARTESIAN_POINT('',(26.5,3.2,0.));
#17225=CARTESIAN_POINT('',(26.5,-3.2,2.4));
#17226=CARTESIAN_POINT('',(26.5,-3.2,2.4));
#17227=CARTESIAN_POINT('Origin',(26.2,0.,2.4));
#17228=CARTESIAN_POINT('',(25.9,3.2,2.4));
#17229=CARTESIAN_POINT('',(26.5,3.2,2.4));
#17230=CARTESIAN_POINT('',(25.9,3.2,2.4));
#17231=CARTESIAN_POINT('Origin',(26.2,0.,2.4));
#17232=CARTESIAN_POINT('',(25.9,-3.2,2.4));
#17233=CARTESIAN_POINT('',(25.9,3.2,2.4));
#17234=CARTESIAN_POINT('',(25.9,-3.2,2.4));
#17235=CARTESIAN_POINT('Origin',(26.2,0.,2.4));
#17236=CARTESIAN_POINT('',(25.9,3.2,2.4));
#17237=CARTESIAN_POINT('Origin',(26.2,-2.5,-0.1));
#17238=CARTESIAN_POINT('',(25.975,-2.5,0.));
#17239=CARTESIAN_POINT('Origin',(26.2,-2.5,0.));
#17240=CARTESIAN_POINT('',(25.975,-2.5,-0.1));
#17241=CARTESIAN_POINT('Origin',(26.2,2.5,-0.1));
#17242=CARTESIAN_POINT('',(25.975,2.5,0.));
#17243=CARTESIAN_POINT('Origin',(26.2,2.5,0.));
#17244=CARTESIAN_POINT('',(25.975,2.5,-0.1));
#17245=CARTESIAN_POINT('Origin',(26.6,0.8,-0.1));
#17246=CARTESIAN_POINT('',(25.9,0.8,1.6));
#17247=CARTESIAN_POINT('',(26.6,0.8,1.6));
#17248=CARTESIAN_POINT('',(25.9,0.8,0.));
#17249=CARTESIAN_POINT('',(25.9,0.8,-0.05));
#17250=CARTESIAN_POINT('',(26.4,0.8,0.));
#17251=CARTESIAN_POINT('Origin',(25.8,-0.8,-0.1));
#17252=CARTESIAN_POINT('',(25.9,-0.8,0.));
#17253=CARTESIAN_POINT('',(26.,-0.8,0.));
#17254=CARTESIAN_POINT('',(25.9,-0.8,1.6));
#17255=CARTESIAN_POINT('',(25.9,-0.8,-0.05));
#17256=CARTESIAN_POINT('',(25.8,-0.8,1.6));
#17257=CARTESIAN_POINT('Origin',(26.2,0.,1.6));
#17258=CARTESIAN_POINT('',(25.9,1.6,1.6));
#17259=CARTESIAN_POINT('Origin',(25.9,3.2,0.));
#17260=CARTESIAN_POINT('',(25.9,3.2,0.));
#17261=CARTESIAN_POINT('',(25.9,3.2,0.));
#17262=CARTESIAN_POINT('',(25.9,3.2,0.));
#17263=CARTESIAN_POINT('',(25.9,-3.2,0.));
#17264=CARTESIAN_POINT('',(25.9,3.2,0.));
#17265=CARTESIAN_POINT('',(25.9,-3.2,0.));
#17266=CARTESIAN_POINT('Origin',(26.2,0.,0.));
#17267=CARTESIAN_POINT('',(25.9,-3.2,0.));
#17268=CARTESIAN_POINT('Origin',(26.2,0.,0.));
#17269=CARTESIAN_POINT('',(26.5,3.2,0.));
#17270=CARTESIAN_POINT('Origin',(26.5,3.2,0.));
#17271=CARTESIAN_POINT('Origin',(25.9,-3.2,0.));
#20004=UNCERTAINTY_MEASURE_WITH_UNIT(LENGTH_MEASURE(0.001),#20097,
'DISTANCE_ACCURACY_VALUE',
'Maximum model space distance between geometric entities at asserted c
onnectivities');
#20042=UNCERTAINTY_MEASURE_WITH_UNIT(LENGTH_MEASURE(0.001),#20097,
'DISTANCE_ACCURACY_VALUE',
'Maximum model space distance between geometric entities at asserted c
onnectivities');
#20058=(
GEOMETRIC_REPRESENTATION_CONTEXT(3)
GLOBAL_UNCERTAINTY_ASSIGNED_CONTEXT((#20004))
GLOBAL_UNIT_ASSIGNED_CONTEXT((#20097,#20099,#20100))
REPRESENTATION_CONTEXT('','3D')
);
#20096=(
GEOMETRIC_REPRESENTATION_CONTEXT(3)
GLOBAL_UNCERTAINTY_ASSIGNED_CONTEXT((#20042))
GLOBAL_UNIT_ASSIGNED_CONTEXT((#20097,#20099,#20100))
REPRESENTATION_CONTEXT('','3D')
);
#20097=(
LENGTH_UNIT()
NAMED_UNIT(*)
SI_UNIT(.CENTI.,.METRE.)
);
#20099=(
NAMED_UNIT(*)
PLANE_ANGLE_UNIT()
SI_UNIT($,.RADIAN.)
);
#20100=(
NAMED_UNIT(*)
SI_UNIT($,.STERADIAN.)
SOLID_ANGLE_UNIT()
);
#20116=SHAPE_DEFINITION_REPRESENTATION(#20169,#20327);
#20169=PRODUCT_DEFINITION_SHAPE('',$,#20381);
#20327=SHAPE_REPRESENTATION('',(#11883),#20058);
#20365=PRODUCT_DEFINITION_CONTEXT('part definition',#20526,'design');
#20381=PRODUCT_DEFINITION('Travel stop (1)','Travel stop (1)',#20434,#20365);
#20434=PRODUCT_DEFINITION_FORMATION('',$,#20543);
#20526=APPLICATION_CONTEXT(
'Core Data for Automotive Mechanical Design Process');
#20527=PRODUCT_CONTEXT('part definition',#20526,'mechanical');
#20543=PRODUCT('Travel stop (1)','Travel stop (1)','Travel stop (1)',(#20527));
#20630=COLOUR_RGB('Light Blue',0.38,0.62,0.78);
#20631=FILL_AREA_STYLE_COLOUR('',#20630);
#20632=FILL_AREA_STYLE('',(#20631));
#20633=SURFACE_STYLE_FILL_AREA(#20632);
#20634=SURFACE_SIDE_STYLE('',(#20633));
#20635=SURFACE_STYLE_USAGE(.BOTH.,#20634);
#20636=PRESENTATION_STYLE_ASSIGNMENT((#20635));
ENDSEC;
END-ISO-10303-21;
